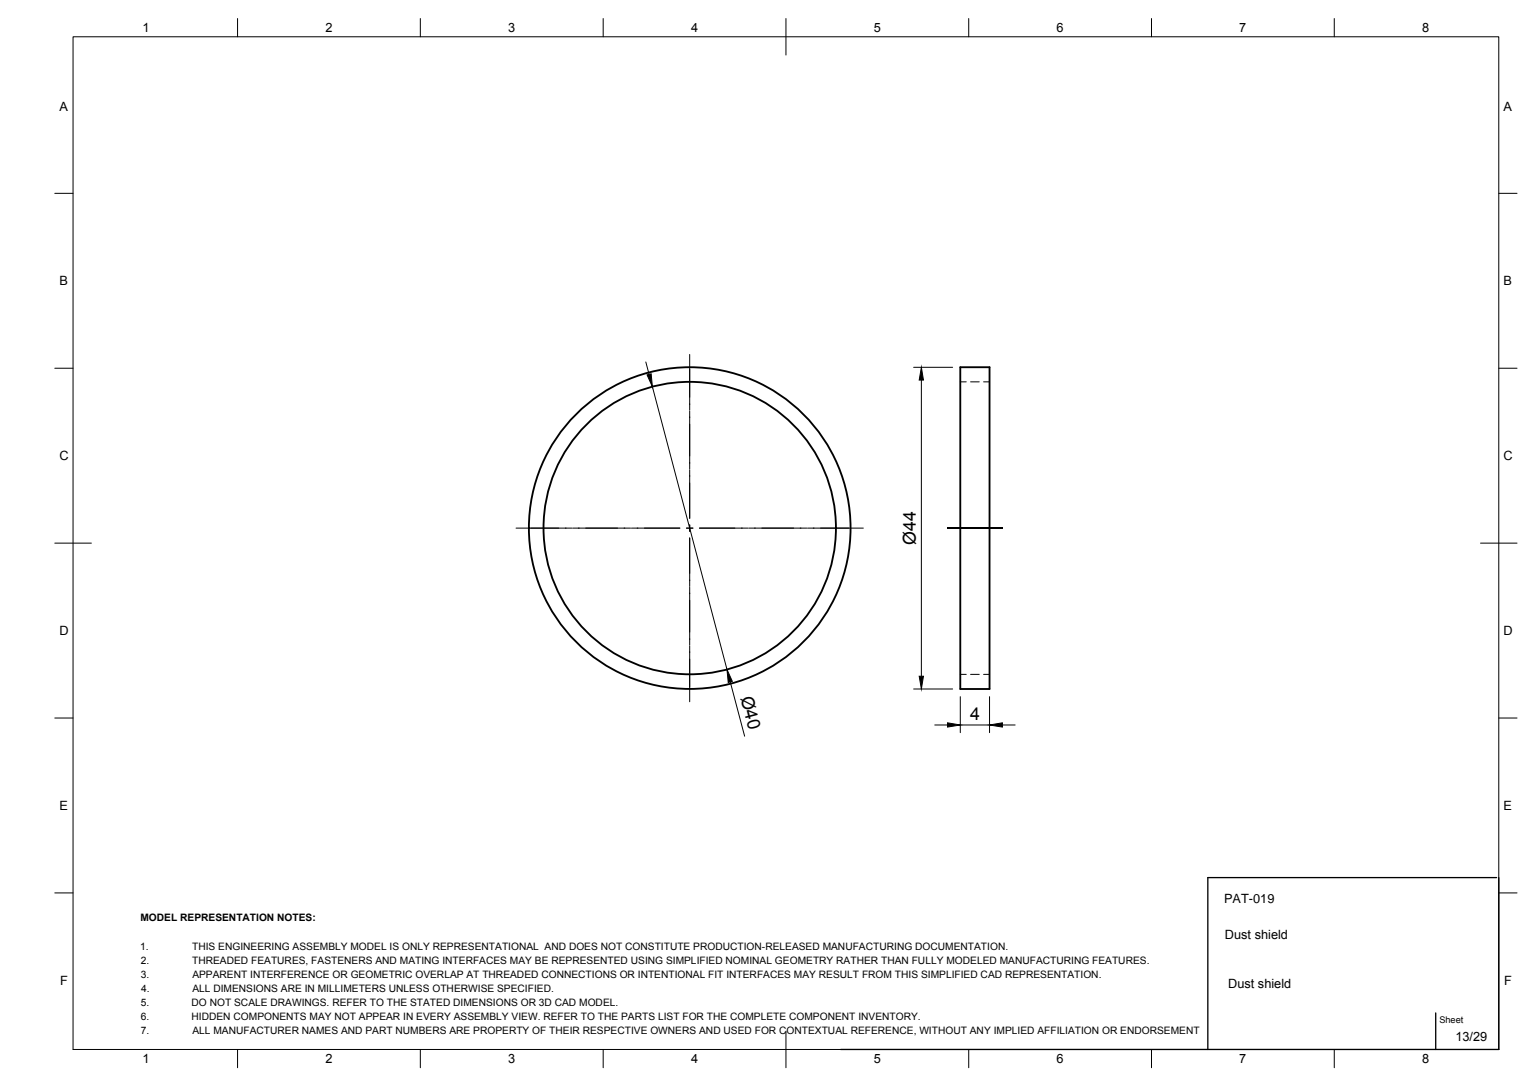
ISO-10303-21;
HEADER;
/* Generated by software containing ST-Developer
 * from STEP Tools, Inc. (www.steptools.com) 
 */

FILE_DESCRIPTION(
/* description */ ('Caster wheel assembly'),
/* implementation_level */ '2;1');

FILE_NAME(
/* name */ 'Dust shield.step',
/* time_stamp */ '2026-10-28T03:23:56-07:00',
/* author */ (''),
/* organization */ (''),
/* preprocessor_version */ 'ST-DEVELOPER v20.2',
/* originating_system */ 'Autodesk Translation Framework v15.17.0.0',
/* authorisation */ '');

FILE_SCHEMA (('AUTOMOTIVE_DESIGN { 1 0 10303 214 3 1 1 }'));
ENDSEC;

DATA;
#10=MECHANICAL_DESIGN_GEOMETRIC_PRESENTATION_REPRESENTATION('',(#230),#5385);
#186=SHAPE_REPRESENTATION_RELATIONSHIP('SRR','None',#5482,#208);
#208=ADVANCED_BREP_SHAPE_REPRESENTATION('',(#260),#5369);
#230=STYLED_ITEM('',(#5686),#260);
#260=MANIFOLD_SOLID_BREP('Body1',#2657);
#305=FACE_BOUND('',#678,.T.);
#306=FACE_BOUND('',#680,.T.);
#373=PLANE('',#3050);
#374=PLANE('',#3051);
#483=FACE_OUTER_BOUND('',#675,.T.);
#484=FACE_OUTER_BOUND('',#676,.T.);
#485=FACE_OUTER_BOUND('',#677,.T.);
#486=FACE_OUTER_BOUND('',#679,.T.);
#675=EDGE_LOOP('',(#2042,#2043,#2044,#2045));
#676=EDGE_LOOP('',(#2046,#2047,#2048,#2049));
#677=EDGE_LOOP('',(#2050));
#678=EDGE_LOOP('',(#2051));
#679=EDGE_LOOP('',(#2052));
#680=EDGE_LOOP('',(#2053));
#885=LINE('',#4523,#1019);
#886=LINE('',#4529,#1020);
#1019=VECTOR('',#3626,2.);
#1020=VECTOR('',#3633,2.2);
#1119=CIRCLE('',#3045,2.);
#1120=CIRCLE('',#3046,2.);
#1121=CIRCLE('',#3048,2.2);
#1122=CIRCLE('',#3049,2.2);
#1322=VERTEX_POINT('',#4520);
#1323=VERTEX_POINT('',#4522);
#1324=VERTEX_POINT('',#4526);
#1325=VERTEX_POINT('',#4528);
#1589=EDGE_CURVE('',#1322,#1322,#1119,.T.);
#1590=EDGE_CURVE('',#1322,#1323,#885,.T.);
#1591=EDGE_CURVE('',#1323,#1323,#1120,.T.);
#1592=EDGE_CURVE('',#1324,#1324,#1121,.T.);
#1593=EDGE_CURVE('',#1324,#1325,#886,.T.);
#1594=EDGE_CURVE('',#1325,#1325,#1122,.T.);
#2042=ORIENTED_EDGE('',*,*,#1589,.F.);
#2043=ORIENTED_EDGE('',*,*,#1590,.T.);
#2044=ORIENTED_EDGE('',*,*,#1591,.T.);
#2045=ORIENTED_EDGE('',*,*,#1590,.F.);
#2046=ORIENTED_EDGE('',*,*,#1592,.F.);
#2047=ORIENTED_EDGE('',*,*,#1593,.T.);
#2048=ORIENTED_EDGE('',*,*,#1594,.T.);
#2049=ORIENTED_EDGE('',*,*,#1593,.F.);
#2050=ORIENTED_EDGE('',*,*,#1592,.T.);
#2051=ORIENTED_EDGE('',*,*,#1589,.T.);
#2052=ORIENTED_EDGE('',*,*,#1594,.F.);
#2053=ORIENTED_EDGE('',*,*,#1591,.F.);
#2448=CYLINDRICAL_SURFACE('',#3044,2.);
#2449=CYLINDRICAL_SURFACE('',#3047,2.2);
#2543=ADVANCED_FACE('',(#483),#2448,.F.);
#2544=ADVANCED_FACE('',(#484),#2449,.T.);
#2545=ADVANCED_FACE('',(#485,#305),#373,.T.);
#2546=ADVANCED_FACE('',(#486,#306),#374,.F.);
#2657=CLOSED_SHELL('',(#2543,#2544,#2545,#2546));
#3043=AXIS2_PLACEMENT_3D('',#4518,#3620,#3621);
#3044=AXIS2_PLACEMENT_3D('',#4519,#3622,#3623);
#3045=AXIS2_PLACEMENT_3D('',#4521,#3624,#3625);
#3046=AXIS2_PLACEMENT_3D('',#4524,#3627,#3628);
#3047=AXIS2_PLACEMENT_3D('',#4525,#3629,#3630);
#3048=AXIS2_PLACEMENT_3D('',#4527,#3631,#3632);
#3049=AXIS2_PLACEMENT_3D('',#4530,#3634,#3635);
#3050=AXIS2_PLACEMENT_3D('',#4531,#3636,#3637);
#3051=AXIS2_PLACEMENT_3D('',#4532,#3638,#3639);
#3620=DIRECTION('axis',(0.,0.,1.));
#3621=DIRECTION('refdir',(1.,0.,0.));
#3622=DIRECTION('center_axis',(0.,0.,1.));
#3623=DIRECTION('ref_axis',(1.,0.,0.));
#3624=DIRECTION('center_axis',(0.,0.,-1.));
#3625=DIRECTION('ref_axis',(1.,0.,0.));
#3626=DIRECTION('',(0.,0.,-1.));
#3627=DIRECTION('center_axis',(0.,0.,-1.));
#3628=DIRECTION('ref_axis',(1.,0.,0.));
#3629=DIRECTION('center_axis',(0.,0.,1.));
#3630=DIRECTION('ref_axis',(1.,0.,0.));
#3631=DIRECTION('center_axis',(0.,0.,1.));
#3632=DIRECTION('ref_axis',(1.,0.,0.));
#3633=DIRECTION('',(0.,0.,-1.));
#3634=DIRECTION('center_axis',(0.,0.,1.));
#3635=DIRECTION('ref_axis',(1.,0.,0.));
#3636=DIRECTION('center_axis',(0.,0.,1.));
#3637=DIRECTION('ref_axis',(1.,0.,0.));
#3638=DIRECTION('center_axis',(0.,0.,1.));
#3639=DIRECTION('ref_axis',(1.,0.,0.));
#4518=CARTESIAN_POINT('',(0.,0.,0.));
#4519=CARTESIAN_POINT('Origin',(-2.,0.,9.3));
#4520=CARTESIAN_POINT('',(-4.,-2.44929359829471E-16,9.7));
#4521=CARTESIAN_POINT('Origin',(-2.,0.,9.7));
#4522=CARTESIAN_POINT('',(-4.,-2.44929359829471E-16,9.3));
#4523=CARTESIAN_POINT('',(-4.,-2.44929359829471E-16,9.3));
#4524=CARTESIAN_POINT('Origin',(-2.,0.,9.3));
#4525=CARTESIAN_POINT('Origin',(-2.,0.,9.3));
#4526=CARTESIAN_POINT('',(-4.2,-2.69422295812418E-16,9.7));
#4527=CARTESIAN_POINT('Origin',(-2.,0.,9.7));
#4528=CARTESIAN_POINT('',(-4.2,-2.69422295812418E-16,9.3));
#4529=CARTESIAN_POINT('',(-4.2,-2.69422295812418E-16,9.3));
#4530=CARTESIAN_POINT('Origin',(-2.,0.,9.3));
#4531=CARTESIAN_POINT('Origin',(-2.,0.,9.7));
#4532=CARTESIAN_POINT('Origin',(-2.,0.,9.3));
#5341=UNCERTAINTY_MEASURE_WITH_UNIT(LENGTH_MEASURE(0.001),#5386,
'DISTANCE_ACCURACY_VALUE',
'Maximum model space distance between geometric entities at asserted c
onnectivities');
#5357=UNCERTAINTY_MEASURE_WITH_UNIT(LENGTH_MEASURE(0.001),#5386,
'DISTANCE_ACCURACY_VALUE',
'Maximum model space distance between geometric entities at asserted c
onnectivities');
#5369=(
GEOMETRIC_REPRESENTATION_CONTEXT(3)
GLOBAL_UNCERTAINTY_ASSIGNED_CONTEXT((#5341))
GLOBAL_UNIT_ASSIGNED_CONTEXT((#5386,#5388,#5389))
REPRESENTATION_CONTEXT('','3D')
);
#5385=(
GEOMETRIC_REPRESENTATION_CONTEXT(3)
GLOBAL_UNCERTAINTY_ASSIGNED_CONTEXT((#5357))
GLOBAL_UNIT_ASSIGNED_CONTEXT((#5386,#5388,#5389))
REPRESENTATION_CONTEXT('','3D')
);
#5386=(
LENGTH_UNIT()
NAMED_UNIT(*)
SI_UNIT(.CENTI.,.METRE.)
);
#5388=(
NAMED_UNIT(*)
PLANE_ANGLE_UNIT()
SI_UNIT($,.RADIAN.)
);
#5389=(
NAMED_UNIT(*)
SI_UNIT($,.STERADIAN.)
SOLID_ANGLE_UNIT()
);
#5401=SHAPE_DEFINITION_REPRESENTATION(#5433,#5482);
#5433=PRODUCT_DEFINITION_SHAPE('',$,#5510);
#5482=SHAPE_REPRESENTATION('',(#3043),#5369);
#5498=PRODUCT_DEFINITION_CONTEXT('part definition',#5581,'design');
#5510=PRODUCT_DEFINITION('Dust shield','Dust shield',#5537,#5498);
#5537=PRODUCT_DEFINITION_FORMATION('',$,#5594);
#5581=APPLICATION_CONTEXT(
'Core Data for Automotive Mechanical Design Process');
#5582=PRODUCT_CONTEXT('part definition',#5581,'mechanical');
#5594=PRODUCT('Dust shield','Dust shield','Dust shield',(#5582));
#5680=COLOUR_RGB('Off White',0.89,0.88,0.83);
#5681=FILL_AREA_STYLE_COLOUR('',#5680);
#5682=FILL_AREA_STYLE('',(#5681));
#5683=SURFACE_STYLE_FILL_AREA(#5682);
#5684=SURFACE_SIDE_STYLE('',(#5683));
#5685=SURFACE_STYLE_USAGE(.BOTH.,#5684);
#5686=PRESENTATION_STYLE_ASSIGNMENT((#5685));
ENDSEC;
END-ISO-10303-21;
